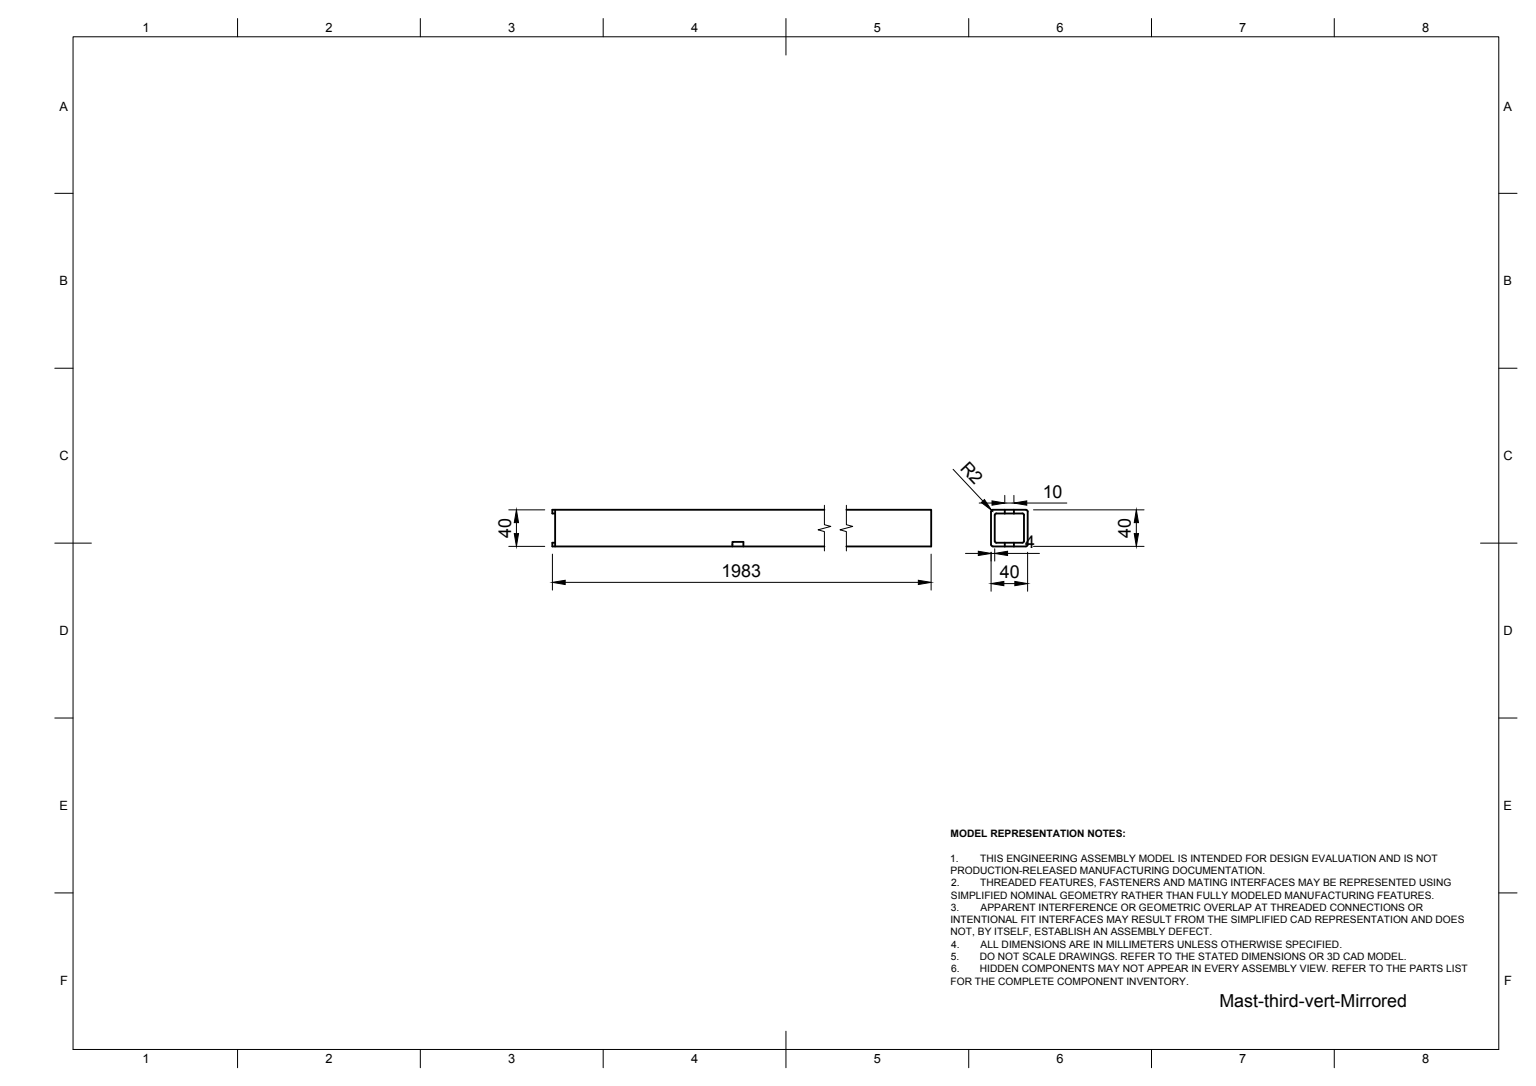
ISO-10303-21;
HEADER;
/* Generated by software containing ST-Developer
 * from STEP Tools, Inc. (www.steptools.com) 
 */

FILE_DESCRIPTION(
/* description */ (''),
/* implementation_level */ '2;1');

FILE_NAME(
/* name */ 'Mast-third-vert-Mirrored.step',
/* time_stamp */ '2026-10-07T11:02:43-07:00',
/* author */ (''),
/* organization */ (''),
/* preprocessor_version */ 'ST-DEVELOPER v20.2',
/* originating_system */ 'Autodesk Translation Framework v15.15.0.0',
/* authorisation */ '');

FILE_SCHEMA (('AUTOMOTIVE_DESIGN { 1 0 10303 214 3 1 1 }'));
ENDSEC;

DATA;
#10=MECHANICAL_DESIGN_GEOMETRIC_PRESENTATION_REPRESENTATION('',(#70),#5505);
#56=SHAPE_REPRESENTATION_RELATIONSHIP('SRR','None',#5541,#63);
#63=ADVANCED_BREP_SHAPE_REPRESENTATION('',(#77),#5502);
#70=STYLED_ITEM('',(#5585),#77);
#77=MANIFOLD_SOLID_BREP('Body1',#3297);
#102=FACE_BOUND('',#532,.T.);
#133=CYLINDRICAL_SURFACE('',#3531,2.);
#134=CYLINDRICAL_SURFACE('',#3535,2.);
#135=CYLINDRICAL_SURFACE('',#3538,1.8);
#136=CYLINDRICAL_SURFACE('',#3541,1.8);
#137=CYLINDRICAL_SURFACE('',#3544,1.8);
#138=CYLINDRICAL_SURFACE('',#3547,1.8);
#139=CYLINDRICAL_SURFACE('',#3553,2.);
#140=CYLINDRICAL_SURFACE('',#3556,2.);
#141=CYLINDRICAL_SURFACE('',#3558,2.);
#142=CYLINDRICAL_SURFACE('',#3559,2.);
#196=CIRCLE('',#3521,1.8);
#197=CIRCLE('',#3522,1.8);
#198=CIRCLE('',#3523,2.);
#199=CIRCLE('',#3524,2.);
#200=CIRCLE('',#3526,2.);
#201=CIRCLE('',#3527,2.);
#202=CIRCLE('',#3528,1.8);
#203=CIRCLE('',#3529,1.8);
#204=CIRCLE('',#3532,2.);
#205=CIRCLE('',#3533,2.);
#206=CIRCLE('',#3536,2.);
#207=CIRCLE('',#3539,1.8);
#208=CIRCLE('',#3542,1.8);
#209=CIRCLE('',#3545,1.8);
#210=CIRCLE('',#3548,1.8);
#211=CIRCLE('',#3550,2.);
#212=CIRCLE('',#3551,2.);
#213=CIRCLE('',#3552,2.);
#214=CIRCLE('',#3554,2.);
#215=CIRCLE('',#3560,2.);
#329=FACE_OUTER_BOUND('',#517,.T.);
#330=FACE_OUTER_BOUND('',#518,.T.);
#331=FACE_OUTER_BOUND('',#519,.T.);
#332=FACE_OUTER_BOUND('',#520,.T.);
#333=FACE_OUTER_BOUND('',#521,.T.);
#334=FACE_OUTER_BOUND('',#522,.T.);
#335=FACE_OUTER_BOUND('',#523,.T.);
#336=FACE_OUTER_BOUND('',#524,.T.);
#337=FACE_OUTER_BOUND('',#525,.T.);
#338=FACE_OUTER_BOUND('',#526,.T.);
#339=FACE_OUTER_BOUND('',#527,.T.);
#340=FACE_OUTER_BOUND('',#528,.T.);
#341=FACE_OUTER_BOUND('',#529,.T.);
#342=FACE_OUTER_BOUND('',#530,.T.);
#343=FACE_OUTER_BOUND('',#531,.T.);
#344=FACE_OUTER_BOUND('',#533,.T.);
#345=FACE_OUTER_BOUND('',#534,.T.);
#346=FACE_OUTER_BOUND('',#535,.T.);
#347=FACE_OUTER_BOUND('',#536,.T.);
#348=FACE_OUTER_BOUND('',#537,.T.);
#349=FACE_OUTER_BOUND('',#538,.T.);
#350=FACE_OUTER_BOUND('',#539,.T.);
#351=FACE_OUTER_BOUND('',#540,.T.);
#352=FACE_OUTER_BOUND('',#541,.T.);
#353=FACE_OUTER_BOUND('',#542,.T.);
#354=FACE_OUTER_BOUND('',#543,.T.);
#355=FACE_OUTER_BOUND('',#544,.T.);
#356=FACE_OUTER_BOUND('',#545,.T.);
#357=FACE_OUTER_BOUND('',#546,.T.);
#358=FACE_OUTER_BOUND('',#547,.T.);
#359=FACE_OUTER_BOUND('',#548,.T.);
#360=FACE_OUTER_BOUND('',#549,.T.);
#361=FACE_OUTER_BOUND('',#550,.T.);
#362=FACE_OUTER_BOUND('',#551,.T.);
#363=FACE_OUTER_BOUND('',#552,.T.);
#517=EDGE_LOOP('',(#2606,#2607,#2608,#2609,#2610,#2611,#2612,#2613,#2614,
#2615,#2616,#2617));
#518=EDGE_LOOP('',(#2618,#2619,#2620,#2621,#2622,#2623,#2624,#2625,#2626,
#2627,#2628,#2629));
#519=EDGE_LOOP('',(#2630,#2631,#2632,#2633,#2634,#2635,#2636,#2637));
#520=EDGE_LOOP('',(#2638,#2639,#2640,#2641));
#521=EDGE_LOOP('',(#2642,#2643,#2644,#2645,#2646,#2647,#2648,#2649,#2650,
#2651,#2652,#2653,#2654,#2655,#2656,#2657));
#522=EDGE_LOOP('',(#2658,#2659,#2660,#2661));
#523=EDGE_LOOP('',(#2662,#2663,#2664,#2665,#2666,#2667,#2668,#2669));
#524=EDGE_LOOP('',(#2670,#2671,#2672,#2673));
#525=EDGE_LOOP('',(#2674,#2675,#2676,#2677));
#526=EDGE_LOOP('',(#2678,#2679,#2680,#2681));
#527=EDGE_LOOP('',(#2682,#2683,#2684,#2685,#2686,#2687,#2688,#2689));
#528=EDGE_LOOP('',(#2690,#2691,#2692,#2693));
#529=EDGE_LOOP('',(#2694,#2695,#2696,#2697));
#530=EDGE_LOOP('',(#2698,#2699,#2700,#2701));
#531=EDGE_LOOP('',(#2702,#2703,#2704,#2705,#2706,#2707,#2708,#2709));
#532=EDGE_LOOP('',(#2710,#2711,#2712,#2713,#2714,#2715,#2716,#2717));
#533=EDGE_LOOP('',(#2718,#2719,#2720,#2721));
#534=EDGE_LOOP('',(#2722,#2723,#2724,#2725,#2726,#2727,#2728,#2729));
#535=EDGE_LOOP('',(#2730,#2731,#2732,#2733));
#536=EDGE_LOOP('',(#2734,#2735,#2736,#2737,#2738,#2739,#2740,#2741));
#537=EDGE_LOOP('',(#2742,#2743,#2744,#2745));
#538=EDGE_LOOP('',(#2746,#2747,#2748,#2749));
#539=EDGE_LOOP('',(#2750,#2751,#2752,#2753,#2754));
#540=EDGE_LOOP('',(#2755,#2756,#2757,#2758));
#541=EDGE_LOOP('',(#2759,#2760,#2761,#2762,#2763));
#542=EDGE_LOOP('',(#2764,#2765,#2766,#2767));
#543=EDGE_LOOP('',(#2768,#2769,#2770,#2771,#2772));
#544=EDGE_LOOP('',(#2773,#2774,#2775,#2776));
#545=EDGE_LOOP('',(#2777,#2778,#2779,#2780,#2781));
#546=EDGE_LOOP('',(#2782,#2783,#2784,#2785));
#547=EDGE_LOOP('',(#2786,#2787,#2788,#2789));
#548=EDGE_LOOP('',(#2790,#2791,#2792,#2793));
#549=EDGE_LOOP('',(#2794,#2795,#2796,#2797));
#550=EDGE_LOOP('',(#2798,#2799,#2800,#2801));
#551=EDGE_LOOP('',(#2802,#2803,#2804,#2805));
#552=EDGE_LOOP('',(#2806,#2807,#2808,#2809));
#813=LINE('',#5076,#1183);
#814=LINE('',#5078,#1184);
#815=LINE('',#5082,#1185);
#816=LINE('',#5086,#1186);
#817=LINE('',#5088,#1187);
#818=LINE('',#5090,#1188);
#819=LINE('',#5094,#1189);
#820=LINE('',#5097,#1190);
#821=LINE('',#5101,#1191);
#822=LINE('',#5105,#1192);
#823=LINE('',#5109,#1193);
#824=LINE('',#5111,#1194);
#825=LINE('',#5113,#1195);
#826=LINE('',#5117,#1196);
#827=LINE('',#5121,#1197);
#828=LINE('',#5122,#1198);
#829=LINE('',#5126,#1199);
#830=LINE('',#5128,#1200);
#831=LINE('',#5129,#1201);
#832=LINE('',#5131,#1202);
#833=LINE('',#5133,#1203);
#834=LINE('',#5135,#1204);
#835=LINE('',#5136,#1205);
#836=LINE('',#5141,#1206);
#837=LINE('',#5145,#1207);
#838=LINE('',#5147,#1208);
#839=LINE('',#5149,#1209);
#840=LINE('',#5151,#1210);
#841=LINE('',#5153,#1211);
#842=LINE('',#5154,#1212);
#843=LINE('',#5156,#1213);
#844=LINE('',#5158,#1214);
#845=LINE('',#5159,#1215);
#846=LINE('',#5161,#1216);
#847=LINE('',#5163,#1217);
#848=LINE('',#5165,#1218);
#849=LINE('',#5166,#1219);
#850=LINE('',#5169,#1220);
#851=LINE('',#5173,#1221);
#852=LINE('',#5175,#1222);
#853=LINE('',#5177,#1223);
#854=LINE('',#5178,#1224);
#855=LINE('',#5180,#1225);
#856=LINE('',#5181,#1226);
#857=LINE('',#5184,#1227);
#858=LINE('',#5188,#1228);
#859=LINE('',#5189,#1229);
#860=LINE('',#5192,#1230);
#861=LINE('',#5196,#1231);
#862=LINE('',#5198,#1232);
#863=LINE('',#5200,#1233);
#864=LINE('',#5201,#1234);
#865=LINE('',#5202,#1235);
#866=LINE('',#5205,#1236);
#867=LINE('',#5209,#1237);
#868=LINE('',#5210,#1238);
#869=LINE('',#5216,#1239);
#870=LINE('',#5221,#1240);
#871=LINE('',#5226,#1241);
#872=LINE('',#5229,#1242);
#873=LINE('',#5230,#1243);
#874=LINE('',#5232,#1244);
#875=LINE('',#5233,#1245);
#876=LINE('',#5235,#1246);
#877=LINE('',#5237,#1247);
#878=LINE('',#5239,#1248);
#879=LINE('',#5241,#1249);
#880=LINE('',#5242,#1250);
#881=LINE('',#5248,#1251);
#882=LINE('',#5249,#1252);
#883=LINE('',#5252,#1253);
#884=LINE('',#5253,#1254);
#885=LINE('',#5255,#1255);
#886=LINE('',#5259,#1256);
#887=LINE('',#5260,#1257);
#888=LINE('',#5263,#1258);
#889=LINE('',#5264,#1259);
#890=LINE('',#5266,#1260);
#891=LINE('',#5269,#1261);
#892=LINE('',#5271,#1262);
#893=LINE('',#5274,#1263);
#894=LINE('',#5276,#1264);
#1183=VECTOR('',#4143,1000.);
#1184=VECTOR('',#4144,1000.);
#1185=VECTOR('',#4147,1000.);
#1186=VECTOR('',#4150,1000.);
#1187=VECTOR('',#4151,1000.);
#1188=VECTOR('',#4152,1000.);
#1189=VECTOR('',#4155,1000.);
#1190=VECTOR('',#4158,1000.);
#1191=VECTOR('',#4161,1000.);
#1192=VECTOR('',#4164,1000.);
#1193=VECTOR('',#4167,1000.);
#1194=VECTOR('',#4168,1000.);
#1195=VECTOR('',#4169,1000.);
#1196=VECTOR('',#4172,1000.);
#1197=VECTOR('',#4175,1000.);
#1198=VECTOR('',#4176,1000.);
#1199=VECTOR('',#4179,1000.);
#1200=VECTOR('',#4180,1000.);
#1201=VECTOR('',#4181,1000.);
#1202=VECTOR('',#4182,1000.);
#1203=VECTOR('',#4183,1000.);
#1204=VECTOR('',#4184,1000.);
#1205=VECTOR('',#4185,1000.);
#1206=VECTOR('',#4190,1000.);
#1207=VECTOR('',#4195,1000.);
#1208=VECTOR('',#4196,1000.);
#1209=VECTOR('',#4197,1000.);
#1210=VECTOR('',#4198,1000.);
#1211=VECTOR('',#4199,1000.);
#1212=VECTOR('',#4200,1000.);
#1213=VECTOR('',#4201,1000.);
#1214=VECTOR('',#4202,1000.);
#1215=VECTOR('',#4203,1000.);
#1216=VECTOR('',#4204,1000.);
#1217=VECTOR('',#4205,1000.);
#1218=VECTOR('',#4206,1000.);
#1219=VECTOR('',#4207,1000.);
#1220=VECTOR('',#4210,1000.);
#1221=VECTOR('',#4215,1000.);
#1222=VECTOR('',#4216,1000.);
#1223=VECTOR('',#4217,1000.);
#1224=VECTOR('',#4218,1000.);
#1225=VECTOR('',#4219,1000.);
#1226=VECTOR('',#4220,1000.);
#1227=VECTOR('',#4223,1000.);
#1228=VECTOR('',#4228,1000.);
#1229=VECTOR('',#4229,1000.);
#1230=VECTOR('',#4232,1000.);
#1231=VECTOR('',#4237,1000.);
#1232=VECTOR('',#4238,1000.);
#1233=VECTOR('',#4239,1000.);
#1234=VECTOR('',#4240,1000.);
#1235=VECTOR('',#4241,1000.);
#1236=VECTOR('',#4244,1000.);
#1237=VECTOR('',#4249,1000.);
#1238=VECTOR('',#4250,1000.);
#1239=VECTOR('',#4257,1000.);
#1240=VECTOR('',#4262,1000.);
#1241=VECTOR('',#4269,1000.);
#1242=VECTOR('',#4272,1000.);
#1243=VECTOR('',#4273,1000.);
#1244=VECTOR('',#4274,1000.);
#1245=VECTOR('',#4275,1000.);
#1246=VECTOR('',#4278,1000.);
#1247=VECTOR('',#4281,1000.);
#1248=VECTOR('',#4282,1000.);
#1249=VECTOR('',#4283,1000.);
#1250=VECTOR('',#4284,1000.);
#1251=VECTOR('',#4293,1000.);
#1252=VECTOR('',#4294,1000.);
#1253=VECTOR('',#4297,1000.);
#1254=VECTOR('',#4298,1000.);
#1255=VECTOR('',#4301,1000.);
#1256=VECTOR('',#4306,1000.);
#1257=VECTOR('',#4307,1000.);
#1258=VECTOR('',#4310,1000.);
#1259=VECTOR('',#4311,1000.);
#1260=VECTOR('',#4314,1000.);
#1261=VECTOR('',#4319,1000.);
#1262=VECTOR('',#4322,1000.);
#1263=VECTOR('',#4327,1000.);
#1264=VECTOR('',#4330,1000.);
#1511=VERTEX_POINT('',#5074);
#1512=VERTEX_POINT('',#5075);
#1513=VERTEX_POINT('',#5077);
#1514=VERTEX_POINT('',#5079);
#1515=VERTEX_POINT('',#5081);
#1516=VERTEX_POINT('',#5083);
#1517=VERTEX_POINT('',#5085);
#1518=VERTEX_POINT('',#5087);
#1519=VERTEX_POINT('',#5089);
#1520=VERTEX_POINT('',#5091);
#1521=VERTEX_POINT('',#5093);
#1522=VERTEX_POINT('',#5095);
#1523=VERTEX_POINT('',#5099);
#1524=VERTEX_POINT('',#5100);
#1525=VERTEX_POINT('',#5102);
#1526=VERTEX_POINT('',#5104);
#1527=VERTEX_POINT('',#5106);
#1528=VERTEX_POINT('',#5108);
#1529=VERTEX_POINT('',#5110);
#1530=VERTEX_POINT('',#5112);
#1531=VERTEX_POINT('',#5114);
#1532=VERTEX_POINT('',#5116);
#1533=VERTEX_POINT('',#5118);
#1534=VERTEX_POINT('',#5120);
#1535=VERTEX_POINT('',#5124);
#1536=VERTEX_POINT('',#5125);
#1537=VERTEX_POINT('',#5127);
#1538=VERTEX_POINT('',#5130);
#1539=VERTEX_POINT('',#5132);
#1540=VERTEX_POINT('',#5134);
#1541=VERTEX_POINT('',#5138);
#1542=VERTEX_POINT('',#5140);
#1543=VERTEX_POINT('',#5144);
#1544=VERTEX_POINT('',#5146);
#1545=VERTEX_POINT('',#5148);
#1546=VERTEX_POINT('',#5150);
#1547=VERTEX_POINT('',#5152);
#1548=VERTEX_POINT('',#5155);
#1549=VERTEX_POINT('',#5157);
#1550=VERTEX_POINT('',#5160);
#1551=VERTEX_POINT('',#5162);
#1552=VERTEX_POINT('',#5164);
#1553=VERTEX_POINT('',#5168);
#1554=VERTEX_POINT('',#5172);
#1555=VERTEX_POINT('',#5174);
#1556=VERTEX_POINT('',#5176);
#1557=VERTEX_POINT('',#5179);
#1558=VERTEX_POINT('',#5183);
#1559=VERTEX_POINT('',#5187);
#1560=VERTEX_POINT('',#5191);
#1561=VERTEX_POINT('',#5195);
#1562=VERTEX_POINT('',#5197);
#1563=VERTEX_POINT('',#5199);
#1564=VERTEX_POINT('',#5204);
#1565=VERTEX_POINT('',#5208);
#1566=VERTEX_POINT('',#5214);
#1567=VERTEX_POINT('',#5215);
#1568=VERTEX_POINT('',#5218);
#1569=VERTEX_POINT('',#5220);
#1570=VERTEX_POINT('',#5224);
#1571=VERTEX_POINT('',#5228);
#1572=VERTEX_POINT('',#5231);
#1573=VERTEX_POINT('',#5238);
#1574=VERTEX_POINT('',#5240);
#1575=VERTEX_POINT('',#5247);
#1576=VERTEX_POINT('',#5251);
#1577=VERTEX_POINT('',#5258);
#1578=VERTEX_POINT('',#5262);
#1898=EDGE_CURVE('',#1511,#1512,#813,.T.);
#1899=EDGE_CURVE('',#1512,#1513,#814,.T.);
#1900=EDGE_CURVE('',#1514,#1513,#196,.T.);
#1901=EDGE_CURVE('',#1515,#1514,#815,.T.);
#1902=EDGE_CURVE('',#1516,#1515,#197,.T.);
#1903=EDGE_CURVE('',#1517,#1516,#816,.T.);
#1904=EDGE_CURVE('',#1517,#1518,#817,.T.);
#1905=EDGE_CURVE('',#1518,#1519,#818,.T.);
#1906=EDGE_CURVE('',#1519,#1520,#198,.T.);
#1907=EDGE_CURVE('',#1520,#1521,#819,.T.);
#1908=EDGE_CURVE('',#1521,#1522,#199,.T.);
#1909=EDGE_CURVE('',#1522,#1511,#820,.F.);
#1910=EDGE_CURVE('',#1523,#1524,#821,.F.);
#1911=EDGE_CURVE('',#1524,#1525,#200,.T.);
#1912=EDGE_CURVE('',#1525,#1526,#822,.F.);
#1913=EDGE_CURVE('',#1526,#1527,#201,.T.);
#1914=EDGE_CURVE('',#1527,#1528,#823,.T.);
#1915=EDGE_CURVE('',#1529,#1528,#824,.T.);
#1916=EDGE_CURVE('',#1530,#1529,#825,.T.);
#1917=EDGE_CURVE('',#1531,#1530,#202,.T.);
#1918=EDGE_CURVE('',#1531,#1532,#826,.T.);
#1919=EDGE_CURVE('',#1533,#1532,#203,.T.);
#1920=EDGE_CURVE('',#1533,#1534,#827,.T.);
#1921=EDGE_CURVE('',#1523,#1534,#828,.T.);
#1922=EDGE_CURVE('',#1535,#1536,#829,.T.);
#1923=EDGE_CURVE('',#1535,#1537,#830,.T.);
#1924=EDGE_CURVE('',#1526,#1537,#831,.T.);
#1925=EDGE_CURVE('',#1525,#1538,#832,.T.);
#1926=EDGE_CURVE('',#1538,#1539,#833,.T.);
#1927=EDGE_CURVE('',#1540,#1539,#834,.T.);
#1928=EDGE_CURVE('',#1536,#1540,#835,.T.);
#1929=EDGE_CURVE('',#1539,#1541,#204,.T.);
#1930=EDGE_CURVE('',#1542,#1541,#836,.T.);
#1931=EDGE_CURVE('',#1540,#1542,#205,.F.);
#1932=EDGE_CURVE('',#1541,#1543,#837,.T.);
#1933=EDGE_CURVE('',#1544,#1543,#838,.T.);
#1934=EDGE_CURVE('',#1544,#1545,#839,.T.);
#1935=EDGE_CURVE('',#1545,#1546,#840,.T.);
#1936=EDGE_CURVE('',#1547,#1546,#841,.T.);
#1937=EDGE_CURVE('',#1519,#1547,#842,.T.);
#1938=EDGE_CURVE('',#1548,#1518,#843,.T.);
#1939=EDGE_CURVE('',#1548,#1549,#844,.T.);
#1940=EDGE_CURVE('',#1549,#1528,#845,.T.);
#1941=EDGE_CURVE('',#1527,#1550,#846,.T.);
#1942=EDGE_CURVE('',#1550,#1551,#847,.T.);
#1943=EDGE_CURVE('',#1552,#1551,#848,.T.);
#1944=EDGE_CURVE('',#1542,#1552,#849,.T.);
#1945=EDGE_CURVE('',#1520,#1553,#850,.T.);
#1946=EDGE_CURVE('',#1553,#1547,#206,.F.);
#1947=EDGE_CURVE('',#1513,#1554,#851,.T.);
#1948=EDGE_CURVE('',#1555,#1512,#852,.T.);
#1949=EDGE_CURVE('',#1555,#1556,#853,.T.);
#1950=EDGE_CURVE('',#1556,#1534,#854,.T.);
#1951=EDGE_CURVE('',#1533,#1557,#855,.T.);
#1952=EDGE_CURVE('',#1557,#1554,#856,.T.);
#1953=EDGE_CURVE('',#1514,#1558,#857,.T.);
#1954=EDGE_CURVE('',#1558,#1554,#207,.T.);
#1955=EDGE_CURVE('',#1515,#1559,#858,.T.);
#1956=EDGE_CURVE('',#1559,#1558,#859,.T.);
#1957=EDGE_CURVE('',#1516,#1560,#860,.T.);
#1958=EDGE_CURVE('',#1560,#1559,#208,.T.);
#1959=EDGE_CURVE('',#1530,#1561,#861,.T.);
#1960=EDGE_CURVE('',#1562,#1529,#862,.T.);
#1961=EDGE_CURVE('',#1563,#1562,#863,.T.);
#1962=EDGE_CURVE('',#1563,#1517,#864,.T.);
#1963=EDGE_CURVE('',#1561,#1560,#865,.T.);
#1964=EDGE_CURVE('',#1531,#1564,#866,.T.);
#1965=EDGE_CURVE('',#1564,#1561,#209,.T.);
#1966=EDGE_CURVE('',#1532,#1565,#867,.T.);
#1967=EDGE_CURVE('',#1564,#1565,#868,.T.);
#1968=EDGE_CURVE('',#1557,#1565,#210,.T.);
#1969=EDGE_CURVE('',#1566,#1567,#869,.T.);
#1970=EDGE_CURVE('',#1543,#1566,#211,.T.);
#1971=EDGE_CURVE('',#1568,#1538,#212,.T.);
#1972=EDGE_CURVE('',#1569,#1568,#870,.T.);
#1973=EDGE_CURVE('',#1567,#1569,#213,.T.);
#1974=EDGE_CURVE('',#1570,#1544,#214,.F.);
#1975=EDGE_CURVE('',#1570,#1566,#871,.T.);
#1976=EDGE_CURVE('',#1571,#1570,#872,.T.);
#1977=EDGE_CURVE('',#1521,#1567,#873,.T.);
#1978=EDGE_CURVE('',#1572,#1553,#874,.T.);
#1979=EDGE_CURVE('',#1572,#1571,#875,.T.);
#1980=EDGE_CURVE('',#1522,#1569,#876,.T.);
#1981=EDGE_CURVE('',#1524,#1568,#877,.T.);
#1982=EDGE_CURVE('',#1573,#1523,#878,.T.);
#1983=EDGE_CURVE('',#1574,#1573,#879,.T.);
#1984=EDGE_CURVE('',#1574,#1511,#880,.T.);
#1985=EDGE_CURVE('',#1537,#1550,#215,.F.);
#1986=EDGE_CURVE('',#1575,#1571,#881,.T.);
#1987=EDGE_CURVE('',#1575,#1545,#882,.T.);
#1988=EDGE_CURVE('',#1576,#1572,#883,.T.);
#1989=EDGE_CURVE('',#1576,#1575,#884,.T.);
#1990=EDGE_CURVE('',#1576,#1546,#885,.T.);
#1991=EDGE_CURVE('',#1577,#1552,#886,.T.);
#1992=EDGE_CURVE('',#1577,#1536,#887,.T.);
#1993=EDGE_CURVE('',#1578,#1577,#888,.T.);
#1994=EDGE_CURVE('',#1578,#1535,#889,.T.);
#1995=EDGE_CURVE('',#1578,#1551,#890,.T.);
#1996=EDGE_CURVE('',#1563,#1548,#891,.T.);
#1997=EDGE_CURVE('',#1562,#1549,#892,.T.);
#1998=EDGE_CURVE('',#1574,#1555,#893,.T.);
#1999=EDGE_CURVE('',#1573,#1556,#894,.T.);
#2606=ORIENTED_EDGE('',*,*,#1898,.T.);
#2607=ORIENTED_EDGE('',*,*,#1899,.T.);
#2608=ORIENTED_EDGE('',*,*,#1900,.F.);
#2609=ORIENTED_EDGE('',*,*,#1901,.F.);
#2610=ORIENTED_EDGE('',*,*,#1902,.F.);
#2611=ORIENTED_EDGE('',*,*,#1903,.F.);
#2612=ORIENTED_EDGE('',*,*,#1904,.T.);
#2613=ORIENTED_EDGE('',*,*,#1905,.T.);
#2614=ORIENTED_EDGE('',*,*,#1906,.T.);
#2615=ORIENTED_EDGE('',*,*,#1907,.T.);
#2616=ORIENTED_EDGE('',*,*,#1908,.T.);
#2617=ORIENTED_EDGE('',*,*,#1909,.T.);
#2618=ORIENTED_EDGE('',*,*,#1910,.T.);
#2619=ORIENTED_EDGE('',*,*,#1911,.T.);
#2620=ORIENTED_EDGE('',*,*,#1912,.T.);
#2621=ORIENTED_EDGE('',*,*,#1913,.T.);
#2622=ORIENTED_EDGE('',*,*,#1914,.T.);
#2623=ORIENTED_EDGE('',*,*,#1915,.F.);
#2624=ORIENTED_EDGE('',*,*,#1916,.F.);
#2625=ORIENTED_EDGE('',*,*,#1917,.F.);
#2626=ORIENTED_EDGE('',*,*,#1918,.T.);
#2627=ORIENTED_EDGE('',*,*,#1919,.F.);
#2628=ORIENTED_EDGE('',*,*,#1920,.T.);
#2629=ORIENTED_EDGE('',*,*,#1921,.F.);
#2630=ORIENTED_EDGE('',*,*,#1922,.F.);
#2631=ORIENTED_EDGE('',*,*,#1923,.T.);
#2632=ORIENTED_EDGE('',*,*,#1924,.F.);
#2633=ORIENTED_EDGE('',*,*,#1912,.F.);
#2634=ORIENTED_EDGE('',*,*,#1925,.T.);
#2635=ORIENTED_EDGE('',*,*,#1926,.T.);
#2636=ORIENTED_EDGE('',*,*,#1927,.F.);
#2637=ORIENTED_EDGE('',*,*,#1928,.F.);
#2638=ORIENTED_EDGE('',*,*,#1927,.T.);
#2639=ORIENTED_EDGE('',*,*,#1929,.T.);
#2640=ORIENTED_EDGE('',*,*,#1930,.F.);
#2641=ORIENTED_EDGE('',*,*,#1931,.F.);
#2642=ORIENTED_EDGE('',*,*,#1930,.T.);
#2643=ORIENTED_EDGE('',*,*,#1932,.T.);
#2644=ORIENTED_EDGE('',*,*,#1933,.F.);
#2645=ORIENTED_EDGE('',*,*,#1934,.T.);
#2646=ORIENTED_EDGE('',*,*,#1935,.T.);
#2647=ORIENTED_EDGE('',*,*,#1936,.F.);
#2648=ORIENTED_EDGE('',*,*,#1937,.F.);
#2649=ORIENTED_EDGE('',*,*,#1905,.F.);
#2650=ORIENTED_EDGE('',*,*,#1938,.F.);
#2651=ORIENTED_EDGE('',*,*,#1939,.T.);
#2652=ORIENTED_EDGE('',*,*,#1940,.T.);
#2653=ORIENTED_EDGE('',*,*,#1914,.F.);
#2654=ORIENTED_EDGE('',*,*,#1941,.T.);
#2655=ORIENTED_EDGE('',*,*,#1942,.T.);
#2656=ORIENTED_EDGE('',*,*,#1943,.F.);
#2657=ORIENTED_EDGE('',*,*,#1944,.F.);
#2658=ORIENTED_EDGE('',*,*,#1945,.F.);
#2659=ORIENTED_EDGE('',*,*,#1906,.F.);
#2660=ORIENTED_EDGE('',*,*,#1937,.T.);
#2661=ORIENTED_EDGE('',*,*,#1946,.F.);
#2662=ORIENTED_EDGE('',*,*,#1947,.F.);
#2663=ORIENTED_EDGE('',*,*,#1899,.F.);
#2664=ORIENTED_EDGE('',*,*,#1948,.F.);
#2665=ORIENTED_EDGE('',*,*,#1949,.T.);
#2666=ORIENTED_EDGE('',*,*,#1950,.T.);
#2667=ORIENTED_EDGE('',*,*,#1920,.F.);
#2668=ORIENTED_EDGE('',*,*,#1951,.T.);
#2669=ORIENTED_EDGE('',*,*,#1952,.T.);
#2670=ORIENTED_EDGE('',*,*,#1953,.F.);
#2671=ORIENTED_EDGE('',*,*,#1900,.T.);
#2672=ORIENTED_EDGE('',*,*,#1947,.T.);
#2673=ORIENTED_EDGE('',*,*,#1954,.F.);
#2674=ORIENTED_EDGE('',*,*,#1955,.F.);
#2675=ORIENTED_EDGE('',*,*,#1901,.T.);
#2676=ORIENTED_EDGE('',*,*,#1953,.T.);
#2677=ORIENTED_EDGE('',*,*,#1956,.F.);
#2678=ORIENTED_EDGE('',*,*,#1957,.F.);
#2679=ORIENTED_EDGE('',*,*,#1902,.T.);
#2680=ORIENTED_EDGE('',*,*,#1955,.T.);
#2681=ORIENTED_EDGE('',*,*,#1958,.F.);
#2682=ORIENTED_EDGE('',*,*,#1959,.F.);
#2683=ORIENTED_EDGE('',*,*,#1916,.T.);
#2684=ORIENTED_EDGE('',*,*,#1960,.F.);
#2685=ORIENTED_EDGE('',*,*,#1961,.F.);
#2686=ORIENTED_EDGE('',*,*,#1962,.T.);
#2687=ORIENTED_EDGE('',*,*,#1903,.T.);
#2688=ORIENTED_EDGE('',*,*,#1957,.T.);
#2689=ORIENTED_EDGE('',*,*,#1963,.F.);
#2690=ORIENTED_EDGE('',*,*,#1964,.F.);
#2691=ORIENTED_EDGE('',*,*,#1917,.T.);
#2692=ORIENTED_EDGE('',*,*,#1959,.T.);
#2693=ORIENTED_EDGE('',*,*,#1965,.F.);
#2694=ORIENTED_EDGE('',*,*,#1966,.F.);
#2695=ORIENTED_EDGE('',*,*,#1918,.F.);
#2696=ORIENTED_EDGE('',*,*,#1964,.T.);
#2697=ORIENTED_EDGE('',*,*,#1967,.T.);
#2698=ORIENTED_EDGE('',*,*,#1968,.F.);
#2699=ORIENTED_EDGE('',*,*,#1951,.F.);
#2700=ORIENTED_EDGE('',*,*,#1919,.T.);
#2701=ORIENTED_EDGE('',*,*,#1966,.T.);
#2702=ORIENTED_EDGE('',*,*,#1969,.F.);
#2703=ORIENTED_EDGE('',*,*,#1970,.F.);
#2704=ORIENTED_EDGE('',*,*,#1932,.F.);
#2705=ORIENTED_EDGE('',*,*,#1929,.F.);
#2706=ORIENTED_EDGE('',*,*,#1926,.F.);
#2707=ORIENTED_EDGE('',*,*,#1971,.F.);
#2708=ORIENTED_EDGE('',*,*,#1972,.F.);
#2709=ORIENTED_EDGE('',*,*,#1973,.F.);
#2710=ORIENTED_EDGE('',*,*,#1954,.T.);
#2711=ORIENTED_EDGE('',*,*,#1952,.F.);
#2712=ORIENTED_EDGE('',*,*,#1968,.T.);
#2713=ORIENTED_EDGE('',*,*,#1967,.F.);
#2714=ORIENTED_EDGE('',*,*,#1965,.T.);
#2715=ORIENTED_EDGE('',*,*,#1963,.T.);
#2716=ORIENTED_EDGE('',*,*,#1958,.T.);
#2717=ORIENTED_EDGE('',*,*,#1956,.T.);
#2718=ORIENTED_EDGE('',*,*,#1974,.T.);
#2719=ORIENTED_EDGE('',*,*,#1933,.T.);
#2720=ORIENTED_EDGE('',*,*,#1970,.T.);
#2721=ORIENTED_EDGE('',*,*,#1975,.F.);
#2722=ORIENTED_EDGE('',*,*,#1976,.T.);
#2723=ORIENTED_EDGE('',*,*,#1975,.T.);
#2724=ORIENTED_EDGE('',*,*,#1969,.T.);
#2725=ORIENTED_EDGE('',*,*,#1977,.F.);
#2726=ORIENTED_EDGE('',*,*,#1907,.F.);
#2727=ORIENTED_EDGE('',*,*,#1945,.T.);
#2728=ORIENTED_EDGE('',*,*,#1978,.F.);
#2729=ORIENTED_EDGE('',*,*,#1979,.T.);
#2730=ORIENTED_EDGE('',*,*,#1980,.F.);
#2731=ORIENTED_EDGE('',*,*,#1908,.F.);
#2732=ORIENTED_EDGE('',*,*,#1977,.T.);
#2733=ORIENTED_EDGE('',*,*,#1973,.T.);
#2734=ORIENTED_EDGE('',*,*,#1981,.F.);
#2735=ORIENTED_EDGE('',*,*,#1910,.F.);
#2736=ORIENTED_EDGE('',*,*,#1982,.F.);
#2737=ORIENTED_EDGE('',*,*,#1983,.F.);
#2738=ORIENTED_EDGE('',*,*,#1984,.T.);
#2739=ORIENTED_EDGE('',*,*,#1909,.F.);
#2740=ORIENTED_EDGE('',*,*,#1980,.T.);
#2741=ORIENTED_EDGE('',*,*,#1972,.T.);
#2742=ORIENTED_EDGE('',*,*,#1925,.F.);
#2743=ORIENTED_EDGE('',*,*,#1911,.F.);
#2744=ORIENTED_EDGE('',*,*,#1981,.T.);
#2745=ORIENTED_EDGE('',*,*,#1971,.T.);
#2746=ORIENTED_EDGE('',*,*,#1985,.T.);
#2747=ORIENTED_EDGE('',*,*,#1941,.F.);
#2748=ORIENTED_EDGE('',*,*,#1913,.F.);
#2749=ORIENTED_EDGE('',*,*,#1924,.T.);
#2750=ORIENTED_EDGE('',*,*,#1974,.F.);
#2751=ORIENTED_EDGE('',*,*,#1976,.F.);
#2752=ORIENTED_EDGE('',*,*,#1986,.F.);
#2753=ORIENTED_EDGE('',*,*,#1987,.T.);
#2754=ORIENTED_EDGE('',*,*,#1934,.F.);
#2755=ORIENTED_EDGE('',*,*,#1979,.F.);
#2756=ORIENTED_EDGE('',*,*,#1988,.F.);
#2757=ORIENTED_EDGE('',*,*,#1989,.T.);
#2758=ORIENTED_EDGE('',*,*,#1986,.T.);
#2759=ORIENTED_EDGE('',*,*,#1978,.T.);
#2760=ORIENTED_EDGE('',*,*,#1946,.T.);
#2761=ORIENTED_EDGE('',*,*,#1936,.T.);
#2762=ORIENTED_EDGE('',*,*,#1990,.F.);
#2763=ORIENTED_EDGE('',*,*,#1988,.T.);
#2764=ORIENTED_EDGE('',*,*,#1935,.F.);
#2765=ORIENTED_EDGE('',*,*,#1987,.F.);
#2766=ORIENTED_EDGE('',*,*,#1989,.F.);
#2767=ORIENTED_EDGE('',*,*,#1990,.T.);
#2768=ORIENTED_EDGE('',*,*,#1928,.T.);
#2769=ORIENTED_EDGE('',*,*,#1931,.T.);
#2770=ORIENTED_EDGE('',*,*,#1944,.T.);
#2771=ORIENTED_EDGE('',*,*,#1991,.F.);
#2772=ORIENTED_EDGE('',*,*,#1992,.T.);
#2773=ORIENTED_EDGE('',*,*,#1922,.T.);
#2774=ORIENTED_EDGE('',*,*,#1992,.F.);
#2775=ORIENTED_EDGE('',*,*,#1993,.F.);
#2776=ORIENTED_EDGE('',*,*,#1994,.T.);
#2777=ORIENTED_EDGE('',*,*,#1985,.F.);
#2778=ORIENTED_EDGE('',*,*,#1923,.F.);
#2779=ORIENTED_EDGE('',*,*,#1994,.F.);
#2780=ORIENTED_EDGE('',*,*,#1995,.T.);
#2781=ORIENTED_EDGE('',*,*,#1942,.F.);
#2782=ORIENTED_EDGE('',*,*,#1991,.T.);
#2783=ORIENTED_EDGE('',*,*,#1943,.T.);
#2784=ORIENTED_EDGE('',*,*,#1995,.F.);
#2785=ORIENTED_EDGE('',*,*,#1993,.T.);
#2786=ORIENTED_EDGE('',*,*,#1904,.F.);
#2787=ORIENTED_EDGE('',*,*,#1962,.F.);
#2788=ORIENTED_EDGE('',*,*,#1996,.T.);
#2789=ORIENTED_EDGE('',*,*,#1938,.T.);
#2790=ORIENTED_EDGE('',*,*,#1915,.T.);
#2791=ORIENTED_EDGE('',*,*,#1940,.F.);
#2792=ORIENTED_EDGE('',*,*,#1997,.F.);
#2793=ORIENTED_EDGE('',*,*,#1960,.T.);
#2794=ORIENTED_EDGE('',*,*,#1996,.F.);
#2795=ORIENTED_EDGE('',*,*,#1961,.T.);
#2796=ORIENTED_EDGE('',*,*,#1997,.T.);
#2797=ORIENTED_EDGE('',*,*,#1939,.F.);
#2798=ORIENTED_EDGE('',*,*,#1898,.F.);
#2799=ORIENTED_EDGE('',*,*,#1984,.F.);
#2800=ORIENTED_EDGE('',*,*,#1998,.T.);
#2801=ORIENTED_EDGE('',*,*,#1948,.T.);
#2802=ORIENTED_EDGE('',*,*,#1921,.T.);
#2803=ORIENTED_EDGE('',*,*,#1950,.F.);
#2804=ORIENTED_EDGE('',*,*,#1999,.F.);
#2805=ORIENTED_EDGE('',*,*,#1982,.T.);
#2806=ORIENTED_EDGE('',*,*,#1998,.F.);
#2807=ORIENTED_EDGE('',*,*,#1983,.T.);
#2808=ORIENTED_EDGE('',*,*,#1999,.T.);
#2809=ORIENTED_EDGE('',*,*,#1949,.F.);
#3074=PLANE('',#3520);
#3075=PLANE('',#3525);
#3076=PLANE('',#3530);
#3077=PLANE('',#3534);
#3078=PLANE('',#3537);
#3079=PLANE('',#3540);
#3080=PLANE('',#3543);
#3081=PLANE('',#3546);
#3082=PLANE('',#3549);
#3083=PLANE('',#3555);
#3084=PLANE('',#3557);
#3085=PLANE('',#3561);
#3086=PLANE('',#3562);
#3087=PLANE('',#3563);
#3088=PLANE('',#3564);
#3089=PLANE('',#3565);
#3090=PLANE('',#3566);
#3091=PLANE('',#3567);
#3092=PLANE('',#3568);
#3093=PLANE('',#3569);
#3094=PLANE('',#3570);
#3095=PLANE('',#3571);
#3096=PLANE('',#3572);
#3097=PLANE('',#3573);
#3098=PLANE('',#3574);
#3220=ADVANCED_FACE('',(#329),#3074,.F.);
#3221=ADVANCED_FACE('',(#330),#3075,.F.);
#3222=ADVANCED_FACE('',(#331),#3076,.T.);
#3223=ADVANCED_FACE('',(#332),#133,.T.);
#3224=ADVANCED_FACE('',(#333),#3077,.T.);
#3225=ADVANCED_FACE('',(#334),#134,.T.);
#3226=ADVANCED_FACE('',(#335),#3078,.T.);
#3227=ADVANCED_FACE('',(#336),#135,.F.);
#3228=ADVANCED_FACE('',(#337),#3079,.T.);
#3229=ADVANCED_FACE('',(#338),#136,.F.);
#3230=ADVANCED_FACE('',(#339),#3080,.T.);
#3231=ADVANCED_FACE('',(#340),#137,.F.);
#3232=ADVANCED_FACE('',(#341),#3081,.T.);
#3233=ADVANCED_FACE('',(#342),#138,.F.);
#3234=ADVANCED_FACE('',(#343,#102),#3082,.T.);
#3235=ADVANCED_FACE('',(#344),#139,.T.);
#3236=ADVANCED_FACE('',(#345),#3083,.T.);
#3237=ADVANCED_FACE('',(#346),#140,.T.);
#3238=ADVANCED_FACE('',(#347),#3084,.T.);
#3239=ADVANCED_FACE('',(#348),#141,.T.);
#3240=ADVANCED_FACE('',(#349),#142,.T.);
#3241=ADVANCED_FACE('',(#350),#3085,.F.);
#3242=ADVANCED_FACE('',(#351),#3086,.F.);
#3243=ADVANCED_FACE('',(#352),#3087,.T.);
#3244=ADVANCED_FACE('',(#353),#3088,.F.);
#3245=ADVANCED_FACE('',(#354),#3089,.T.);
#3246=ADVANCED_FACE('',(#355),#3090,.T.);
#3247=ADVANCED_FACE('',(#356),#3091,.F.);
#3248=ADVANCED_FACE('',(#357),#3092,.T.);
#3249=ADVANCED_FACE('',(#358),#3093,.F.);
#3250=ADVANCED_FACE('',(#359),#3094,.T.);
#3251=ADVANCED_FACE('',(#360),#3095,.F.);
#3252=ADVANCED_FACE('',(#361),#3096,.F.);
#3253=ADVANCED_FACE('',(#362),#3097,.T.);
#3254=ADVANCED_FACE('',(#363),#3098,.F.);
#3297=CLOSED_SHELL('',(#3220,#3221,#3222,#3223,#3224,#3225,#3226,#3227,
#3228,#3229,#3230,#3231,#3232,#3233,#3234,#3235,#3236,#3237,#3238,#3239,
#3240,#3241,#3242,#3243,#3244,#3245,#3246,#3247,#3248,#3249,#3250,#3251,
#3252,#3253,#3254));
#3519=AXIS2_PLACEMENT_3D('',#5072,#4139,#4140);
#3520=AXIS2_PLACEMENT_3D('',#5073,#4141,#4142);
#3521=AXIS2_PLACEMENT_3D('',#5080,#4145,#4146);
#3522=AXIS2_PLACEMENT_3D('',#5084,#4148,#4149);
#3523=AXIS2_PLACEMENT_3D('',#5092,#4153,#4154);
#3524=AXIS2_PLACEMENT_3D('',#5096,#4156,#4157);
#3525=AXIS2_PLACEMENT_3D('',#5098,#4159,#4160);
#3526=AXIS2_PLACEMENT_3D('',#5103,#4162,#4163);
#3527=AXIS2_PLACEMENT_3D('',#5107,#4165,#4166);
#3528=AXIS2_PLACEMENT_3D('',#5115,#4170,#4171);
#3529=AXIS2_PLACEMENT_3D('',#5119,#4173,#4174);
#3530=AXIS2_PLACEMENT_3D('',#5123,#4177,#4178);
#3531=AXIS2_PLACEMENT_3D('',#5137,#4186,#4187);
#3532=AXIS2_PLACEMENT_3D('',#5139,#4188,#4189);
#3533=AXIS2_PLACEMENT_3D('',#5142,#4191,#4192);
#3534=AXIS2_PLACEMENT_3D('',#5143,#4193,#4194);
#3535=AXIS2_PLACEMENT_3D('',#5167,#4208,#4209);
#3536=AXIS2_PLACEMENT_3D('',#5170,#4211,#4212);
#3537=AXIS2_PLACEMENT_3D('',#5171,#4213,#4214);
#3538=AXIS2_PLACEMENT_3D('',#5182,#4221,#4222);
#3539=AXIS2_PLACEMENT_3D('',#5185,#4224,#4225);
#3540=AXIS2_PLACEMENT_3D('',#5186,#4226,#4227);
#3541=AXIS2_PLACEMENT_3D('',#5190,#4230,#4231);
#3542=AXIS2_PLACEMENT_3D('',#5193,#4233,#4234);
#3543=AXIS2_PLACEMENT_3D('',#5194,#4235,#4236);
#3544=AXIS2_PLACEMENT_3D('',#5203,#4242,#4243);
#3545=AXIS2_PLACEMENT_3D('',#5206,#4245,#4246);
#3546=AXIS2_PLACEMENT_3D('',#5207,#4247,#4248);
#3547=AXIS2_PLACEMENT_3D('',#5211,#4251,#4252);
#3548=AXIS2_PLACEMENT_3D('',#5212,#4253,#4254);
#3549=AXIS2_PLACEMENT_3D('',#5213,#4255,#4256);
#3550=AXIS2_PLACEMENT_3D('',#5217,#4258,#4259);
#3551=AXIS2_PLACEMENT_3D('',#5219,#4260,#4261);
#3552=AXIS2_PLACEMENT_3D('',#5222,#4263,#4264);
#3553=AXIS2_PLACEMENT_3D('',#5223,#4265,#4266);
#3554=AXIS2_PLACEMENT_3D('',#5225,#4267,#4268);
#3555=AXIS2_PLACEMENT_3D('',#5227,#4270,#4271);
#3556=AXIS2_PLACEMENT_3D('',#5234,#4276,#4277);
#3557=AXIS2_PLACEMENT_3D('',#5236,#4279,#4280);
#3558=AXIS2_PLACEMENT_3D('',#5243,#4285,#4286);
#3559=AXIS2_PLACEMENT_3D('',#5244,#4287,#4288);
#3560=AXIS2_PLACEMENT_3D('',#5245,#4289,#4290);
#3561=AXIS2_PLACEMENT_3D('',#5246,#4291,#4292);
#3562=AXIS2_PLACEMENT_3D('',#5250,#4295,#4296);
#3563=AXIS2_PLACEMENT_3D('',#5254,#4299,#4300);
#3564=AXIS2_PLACEMENT_3D('',#5256,#4302,#4303);
#3565=AXIS2_PLACEMENT_3D('',#5257,#4304,#4305);
#3566=AXIS2_PLACEMENT_3D('',#5261,#4308,#4309);
#3567=AXIS2_PLACEMENT_3D('',#5265,#4312,#4313);
#3568=AXIS2_PLACEMENT_3D('',#5267,#4315,#4316);
#3569=AXIS2_PLACEMENT_3D('',#5268,#4317,#4318);
#3570=AXIS2_PLACEMENT_3D('',#5270,#4320,#4321);
#3571=AXIS2_PLACEMENT_3D('',#5272,#4323,#4324);
#3572=AXIS2_PLACEMENT_3D('',#5273,#4325,#4326);
#3573=AXIS2_PLACEMENT_3D('',#5275,#4328,#4329);
#3574=AXIS2_PLACEMENT_3D('',#5277,#4331,#4332);
#4139=DIRECTION('axis',(0.,0.,1.));
#4140=DIRECTION('refdir',(1.,0.,0.));
#4141=DIRECTION('center_axis',(-1.22464679914735E-16,0.,1.));
#4142=DIRECTION('ref_axis',(-1.,0.,-1.22464679914735E-16));
#4143=DIRECTION('',(-1.,1.32329071915687E-32,-2.28847549044393E-17));
#4144=DIRECTION('',(4.88654500275157E-16,1.,5.98429169650921E-32));
#4145=DIRECTION('center_axis',(1.22464679914735E-16,0.,-1.));
#4146=DIRECTION('ref_axis',(0.,-1.,0.));
#4147=DIRECTION('',(1.,-4.88654500275157E-16,1.22464679914735E-16));
#4148=DIRECTION('center_axis',(1.22464679914735E-16,0.,-1.));
#4149=DIRECTION('ref_axis',(0.,-1.,0.));
#4150=DIRECTION('',(4.88654500275157E-16,1.,5.9842916965092E-32));
#4151=DIRECTION('',(-1.,1.32329071915687E-32,-2.28847549044393E-17));
#4152=DIRECTION('',(5.78241158658936E-16,1.,7.08141184086923E-32));
#4153=DIRECTION('center_axis',(1.22464679914735E-16,0.,-1.));
#4154=DIRECTION('ref_axis',(0.,-1.,0.));
#4155=DIRECTION('',(1.,-5.78241158658936E-16,1.22464679914735E-16));
#4156=DIRECTION('center_axis',(1.22464679914735E-16,0.,-1.));
#4157=DIRECTION('ref_axis',(0.,-1.,0.));
#4158=DIRECTION('',(5.78241158658936E-16,1.,7.08141184086923E-32));
#4159=DIRECTION('center_axis',(-1.22464679914735E-16,0.,1.));
#4160=DIRECTION('ref_axis',(-1.,0.,-1.22464679914735E-16));
#4161=DIRECTION('',(5.78241158658936E-16,1.,7.08141184086923E-32));
#4162=DIRECTION('center_axis',(1.22464679914735E-16,0.,-1.));
#4163=DIRECTION('ref_axis',(0.,-1.,0.));
#4164=DIRECTION('',(1.,-5.78241158658936E-16,1.22464679914735E-16));
#4165=DIRECTION('center_axis',(1.22464679914735E-16,0.,-1.));
#4166=DIRECTION('ref_axis',(0.,-1.,0.));
#4167=DIRECTION('',(5.78241158658936E-16,1.,7.08141184086923E-32));
#4168=DIRECTION('',(-1.,1.32329071915687E-32,-2.28847549044393E-17));
#4169=DIRECTION('',(4.88654500275157E-16,1.,5.9842916965092E-32));
#4170=DIRECTION('center_axis',(1.22464679914735E-16,0.,-1.));
#4171=DIRECTION('ref_axis',(0.,-1.,0.));
#4172=DIRECTION('',(1.,0.,1.22464679914735E-16));
#4173=DIRECTION('center_axis',(1.22464679914735E-16,0.,-1.));
#4174=DIRECTION('ref_axis',(0.,-1.,0.));
#4175=DIRECTION('',(4.88654500275157E-16,1.,5.98429169650921E-32));
#4176=DIRECTION('',(-1.,1.32329071915687E-32,-2.28847549044393E-17));
#4177=DIRECTION('center_axis',(-5.78241158658936E-16,-1.,-7.08141184086922E-32));
#4178=DIRECTION('ref_axis',(1.,-5.78241158658936E-16,0.));
#4179=DIRECTION('',(-4.09476378780532E-47,-7.08141184086922E-32,1.));
#4180=DIRECTION('',(-1.,5.78241158658936E-16,4.09476378780532E-47));
#4181=DIRECTION('',(-1.22464679914735E-16,0.,1.));
#4182=DIRECTION('',(-1.22464679914735E-16,0.,1.));
#4183=DIRECTION('',(-1.,5.78241158658936E-16,-3.06161699786839E-16));
#4184=DIRECTION('',(-1.22464679914735E-16,0.,1.));
#4185=DIRECTION('',(-1.,5.78241158658936E-16,4.09476378780532E-47));
#4186=DIRECTION('center_axis',(-1.22464679914735E-16,0.,1.));
#4187=DIRECTION('ref_axis',(-1.,0.,-1.22464679914735E-16));
#4188=DIRECTION('center_axis',(3.06161699786839E-16,0.,-1.));
#4189=DIRECTION('ref_axis',(-1.,0.,-3.06161699786839E-16));
#4190=DIRECTION('',(-1.22464679914735E-16,0.,1.));
#4191=DIRECTION('center_axis',(0.,-7.08141184086922E-32,1.));
#4192=DIRECTION('ref_axis',(0.,-1.,-7.08141184086922E-32));
#4193=DIRECTION('center_axis',(-1.,5.78241158658936E-16,-1.22464679914735E-16));
#4194=DIRECTION('ref_axis',(-5.78241158658936E-16,-1.,-1.41228329145101E-48));
#4195=DIRECTION('',(5.78241158658936E-16,1.,1.77035296021731E-31));
#4196=DIRECTION('',(-1.22464679914735E-16,0.,1.));
#4197=DIRECTION('',(-5.78241158658936E-16,-1.,0.));
#4198=DIRECTION('',(1.22464679914735E-16,-7.08141184086923E-32,-1.));
#4199=DIRECTION('',(-5.78241158658936E-16,-1.,0.));
#4200=DIRECTION('',(-1.22464679914735E-16,0.,1.));
#4201=DIRECTION('',(-2.28847549044393E-17,-5.78241158658936E-16,1.));
#4202=DIRECTION('',(1.32329071915687E-32,-1.,-5.78241158658936E-16));
#4203=DIRECTION('',(-2.28847549044393E-17,-5.78241158658936E-16,1.));
#4204=DIRECTION('',(-1.22464679914735E-16,0.,1.));
#4205=DIRECTION('',(5.78241158658936E-16,1.,7.08141184086922E-32));
#4206=DIRECTION('',(1.22464679914735E-16,-1.09476442525376E-47,-1.));
#4207=DIRECTION('',(5.78241158658936E-16,1.,7.08141184086922E-32));
#4208=DIRECTION('center_axis',(-1.22464679914735E-16,0.,1.));
#4209=DIRECTION('ref_axis',(-1.,0.,-1.22464679914735E-16));
#4210=DIRECTION('',(-1.22464679914735E-16,0.,1.));
#4211=DIRECTION('center_axis',(0.,0.,-1.));
#4212=DIRECTION('ref_axis',(-1.,0.,0.));
#4213=DIRECTION('center_axis',(-1.,4.88654500275157E-16,-1.22464679914735E-16));
#4214=DIRECTION('ref_axis',(-4.88654500275157E-16,-1.,-3.23663765428249E-48));
#4215=DIRECTION('',(-1.22464679914735E-16,0.,1.));
#4216=DIRECTION('',(-2.28847549044393E-17,-5.78241158658936E-16,1.));
#4217=DIRECTION('',(1.32329071915687E-32,-1.,-5.78241158658936E-16));
#4218=DIRECTION('',(-2.28847549044393E-17,-5.78241158658936E-16,1.));
#4219=DIRECTION('',(-1.22464679914735E-16,0.,1.));
#4220=DIRECTION('',(4.88654500275157E-16,1.,1.4960729241273E-31));
#4221=DIRECTION('center_axis',(-1.22464679914735E-16,0.,1.));
#4222=DIRECTION('ref_axis',(-1.,0.,-1.22464679914735E-16));
#4223=DIRECTION('',(-1.22464679914735E-16,0.,1.));
#4224=DIRECTION('center_axis',(3.06161699786839E-16,0.,-1.));
#4225=DIRECTION('ref_axis',(-1.,0.,-3.06161699786839E-16));
#4226=DIRECTION('center_axis',(-4.88654500275157E-16,-1.,-5.9842916965092E-32));
#4227=DIRECTION('ref_axis',(1.,-4.88654500275157E-16,0.));
#4228=DIRECTION('',(-1.22464679914735E-16,0.,1.));
#4229=DIRECTION('',(1.,-4.88654500275157E-16,3.06161699786839E-16));
#4230=DIRECTION('center_axis',(-1.22464679914735E-16,0.,1.));
#4231=DIRECTION('ref_axis',(-1.,0.,-1.22464679914735E-16));
#4232=DIRECTION('',(-1.22464679914735E-16,0.,1.));
#4233=DIRECTION('center_axis',(3.06161699786839E-16,0.,-1.));
#4234=DIRECTION('ref_axis',(-1.,0.,-3.06161699786839E-16));
#4235=DIRECTION('center_axis',(1.,-4.88654500275157E-16,1.22464679914735E-16));
#4236=DIRECTION('ref_axis',(4.88654500275157E-16,1.,3.23663765428249E-48));
#4237=DIRECTION('',(-1.22464679914735E-16,0.,1.));
#4238=DIRECTION('',(-2.28847549044393E-17,-5.78241158658936E-16,1.));
#4239=DIRECTION('',(1.32329071915687E-32,-1.,-5.78241158658936E-16));
#4240=DIRECTION('',(-2.28847549044393E-17,-5.78241158658936E-16,1.));
#4241=DIRECTION('',(4.88654500275157E-16,1.,1.4960729241273E-31));
#4242=DIRECTION('center_axis',(-1.22464679914735E-16,0.,1.));
#4243=DIRECTION('ref_axis',(-1.,0.,-1.22464679914735E-16));
#4244=DIRECTION('',(-1.22464679914735E-16,0.,1.));
#4245=DIRECTION('center_axis',(3.06161699786839E-16,0.,-1.));
#4246=DIRECTION('ref_axis',(-1.,0.,-3.06161699786839E-16));
#4247=DIRECTION('center_axis',(0.,1.,0.));
#4248=DIRECTION('ref_axis',(0.,0.,-1.));
#4249=DIRECTION('',(-1.22464679914735E-16,0.,1.));
#4250=DIRECTION('',(1.,0.,3.06161699786839E-16));
#4251=DIRECTION('center_axis',(-1.22464679914735E-16,0.,1.));
#4252=DIRECTION('ref_axis',(-1.,0.,-1.22464679914735E-16));
#4253=DIRECTION('center_axis',(3.06161699786839E-16,0.,-1.));
#4254=DIRECTION('ref_axis',(-1.,0.,-3.06161699786839E-16));
#4255=DIRECTION('center_axis',(-3.06161699786839E-16,0.,1.));
#4256=DIRECTION('ref_axis',(1.,0.,3.06161699786839E-16));
#4257=DIRECTION('',(1.,-5.78241158658936E-16,3.06161699786839E-16));
#4258=DIRECTION('center_axis',(3.06161699786839E-16,0.,-1.));
#4259=DIRECTION('ref_axis',(-1.,0.,-3.06161699786839E-16));
#4260=DIRECTION('center_axis',(3.06161699786839E-16,0.,-1.));
#4261=DIRECTION('ref_axis',(-1.,0.,-3.06161699786839E-16));
#4262=DIRECTION('',(-5.78241158658936E-16,-1.,-1.77035296021731E-31));
#4263=DIRECTION('center_axis',(3.06161699786839E-16,0.,-1.));
#4264=DIRECTION('ref_axis',(-1.,0.,-3.06161699786839E-16));
#4265=DIRECTION('center_axis',(-1.22464679914735E-16,0.,1.));
#4266=DIRECTION('ref_axis',(-1.,0.,-1.22464679914735E-16));
#4267=DIRECTION('center_axis',(0.,0.,-1.));
#4268=DIRECTION('ref_axis',(-1.,0.,0.));
#4269=DIRECTION('',(-1.22464679914735E-16,0.,1.));
#4270=DIRECTION('center_axis',(5.78241158658936E-16,1.,7.08141184086922E-32));
#4271=DIRECTION('ref_axis',(-1.,5.78241158658936E-16,0.));
#4272=DIRECTION('',(-1.,5.78241158658936E-16,0.));
#4273=DIRECTION('',(-1.22464679914735E-16,0.,1.));
#4274=DIRECTION('',(-1.,5.78241158658936E-16,0.));
#4275=DIRECTION('',(0.,0.,1.));
#4276=DIRECTION('center_axis',(-1.22464679914735E-16,0.,1.));
#4277=DIRECTION('ref_axis',(-1.,0.,-1.22464679914735E-16));
#4278=DIRECTION('',(-1.22464679914735E-16,0.,1.));
#4279=DIRECTION('center_axis',(1.,-5.78241158658936E-16,1.22464679914735E-16));
#4280=DIRECTION('ref_axis',(5.78241158658936E-16,1.,1.41228329145101E-48));
#4281=DIRECTION('',(-1.22464679914735E-16,0.,1.));
#4282=DIRECTION('',(-2.28847549044393E-17,-5.78241158658936E-16,1.));
#4283=DIRECTION('',(1.32329071915687E-32,-1.,-5.78241158658936E-16));
#4284=DIRECTION('',(-2.28847549044393E-17,-5.78241158658936E-16,1.));
#4285=DIRECTION('center_axis',(-1.22464679914735E-16,0.,1.));
#4286=DIRECTION('ref_axis',(-1.,0.,-1.22464679914735E-16));
#4287=DIRECTION('center_axis',(-1.22464679914735E-16,0.,1.));
#4288=DIRECTION('ref_axis',(-1.,0.,-1.22464679914735E-16));
#4289=DIRECTION('center_axis',(0.,-7.08141184086922E-32,1.));
#4290=DIRECTION('ref_axis',(0.,-1.,-7.08141184086922E-32));
#4291=DIRECTION('center_axis',(0.,0.,1.));
#4292=DIRECTION('ref_axis',(-1.,0.,0.));
#4293=DIRECTION('',(5.78241158658936E-16,1.,0.));
#4294=DIRECTION('',(-1.,5.78241158658936E-16,0.));
#4295=DIRECTION('center_axis',(1.,-5.78241158658936E-16,0.));
#4296=DIRECTION('ref_axis',(5.78241158658936E-16,1.,0.));
#4297=DIRECTION('',(5.78241158658936E-16,1.,0.));
#4298=DIRECTION('',(0.,0.,1.));
#4299=DIRECTION('center_axis',(0.,0.,1.));
#4300=DIRECTION('ref_axis',(-1.,0.,0.));
#4301=DIRECTION('',(-1.,5.78241158658936E-16,0.));
#4302=DIRECTION('center_axis',(-5.78241158658936E-16,-1.,0.));
#4303=DIRECTION('ref_axis',(1.,-5.78241158658936E-16,0.));
#4304=DIRECTION('center_axis',(0.,7.08141184086922E-32,-1.));
#4305=DIRECTION('ref_axis',(0.,-1.,-7.08141184086922E-32));
#4306=DIRECTION('',(-1.,5.78241158658936E-16,4.09476378780532E-47));
#4307=DIRECTION('',(-5.78241158658936E-16,-1.,-7.08141184086922E-32));
#4308=DIRECTION('center_axis',(-1.,5.78241158658936E-16,0.));
#4309=DIRECTION('ref_axis',(-5.78241158658936E-16,-1.,0.));
#4310=DIRECTION('',(-4.09476378780532E-47,-7.08141184086922E-32,1.));
#4311=DIRECTION('',(-5.78241158658936E-16,-1.,-7.08141184086922E-32));
#4312=DIRECTION('center_axis',(0.,7.08141184086922E-32,-1.));
#4313=DIRECTION('ref_axis',(0.,-1.,-7.08141184086922E-32));
#4314=DIRECTION('',(-1.,5.78241158658936E-16,4.09476378780532E-47));
#4315=DIRECTION('center_axis',(-5.78241158658936E-16,-1.,-7.08141184086922E-32));
#4316=DIRECTION('ref_axis',(1.,-5.78241158658936E-16,-4.09476378780532E-47));
#4317=DIRECTION('center_axis',(1.78184314006146E-48,-1.,-5.78241158658936E-16));
#4318=DIRECTION('ref_axis',(-6.41902719210046E-80,-5.78241158658936E-16,
1.));
#4319=DIRECTION('',(-1.,1.32329071915687E-32,-2.28847549044393E-17));
#4320=DIRECTION('center_axis',(1.78184314006146E-48,-1.,-5.78241158658936E-16));
#4321=DIRECTION('ref_axis',(-6.41902719210046E-80,-5.78241158658936E-16,
1.));
#4322=DIRECTION('',(-1.,1.32329071915687E-32,-2.28847549044393E-17));
#4323=DIRECTION('center_axis',(-2.28847549044393E-17,-5.78241158658936E-16,
1.));
#4324=DIRECTION('ref_axis',(1.,-1.32329071915687E-32,2.28847549044393E-17));
#4325=DIRECTION('center_axis',(1.78184314006146E-48,-1.,-5.78241158658936E-16));
#4326=DIRECTION('ref_axis',(-6.41902719210046E-80,-5.78241158658936E-16,
1.));
#4327=DIRECTION('',(-1.,1.32329071915687E-32,-2.28847549044393E-17));
#4328=DIRECTION('center_axis',(1.78184314006146E-48,-1.,-5.78241158658936E-16));
#4329=DIRECTION('ref_axis',(-6.41902719210046E-80,-5.78241158658936E-16,
1.));
#4330=DIRECTION('',(-1.,1.32329071915687E-32,-2.28847549044393E-17));
#4331=DIRECTION('center_axis',(-2.28847549044393E-17,-5.78241158658936E-16,
1.));
#4332=DIRECTION('ref_axis',(1.,-1.32329071915687E-32,2.28847549044393E-17));
#5072=CARTESIAN_POINT('',(0.,0.,0.));
#5073=CARTESIAN_POINT('Origin',(-360.,850.,-2152.));
#5074=CARTESIAN_POINT('',(-340.,855.,-2152.));
#5075=CARTESIAN_POINT('',(-344.,855.,-2152.));
#5076=CARTESIAN_POINT('',(-342.,855.,-2152.));
#5077=CARTESIAN_POINT('',(-344.,864.2,-2152.));
#5078=CARTESIAN_POINT('',(-344.,850.,-2152.));
#5079=CARTESIAN_POINT('',(-345.8,866.,-2152.));
#5080=CARTESIAN_POINT('Origin',(-345.8,864.2,-2152.));
#5081=CARTESIAN_POINT('',(-374.2,866.,-2152.));
#5082=CARTESIAN_POINT('',(-360.,866.,-2152.));
#5083=CARTESIAN_POINT('',(-376.,864.2,-2152.));
#5084=CARTESIAN_POINT('Origin',(-374.2,864.2,-2152.));
#5085=CARTESIAN_POINT('',(-376.,855.,-2152.));
#5086=CARTESIAN_POINT('',(-376.,850.,-2152.));
#5087=CARTESIAN_POINT('',(-380.,855.,-2152.));
#5088=CARTESIAN_POINT('',(-378.,855.,-2152.));
#5089=CARTESIAN_POINT('',(-380.,868.,-2152.));
#5090=CARTESIAN_POINT('',(-380.,850.,-2152.));
#5091=CARTESIAN_POINT('',(-378.,870.,-2152.));
#5092=CARTESIAN_POINT('Origin',(-378.,868.,-2152.));
#5093=CARTESIAN_POINT('',(-342.,870.,-2152.));
#5094=CARTESIAN_POINT('',(-360.,870.,-2152.));
#5095=CARTESIAN_POINT('',(-340.,868.,-2152.));
#5096=CARTESIAN_POINT('Origin',(-342.,868.,-2152.));
#5097=CARTESIAN_POINT('',(-340.,850.,-2152.));
#5098=CARTESIAN_POINT('Origin',(-360.,850.,-2152.));
#5099=CARTESIAN_POINT('',(-340.,845.,-2152.));
#5100=CARTESIAN_POINT('',(-340.,832.,-2152.));
#5101=CARTESIAN_POINT('',(-340.,850.,-2152.));
#5102=CARTESIAN_POINT('',(-342.,830.,-2152.));
#5103=CARTESIAN_POINT('Origin',(-342.,832.,-2152.));
#5104=CARTESIAN_POINT('',(-378.,830.,-2152.));
#5105=CARTESIAN_POINT('',(-360.,830.,-2152.));
#5106=CARTESIAN_POINT('',(-380.,832.,-2152.));
#5107=CARTESIAN_POINT('Origin',(-378.,832.,-2152.));
#5108=CARTESIAN_POINT('',(-380.,845.,-2152.));
#5109=CARTESIAN_POINT('',(-380.,850.,-2152.));
#5110=CARTESIAN_POINT('',(-376.,845.,-2152.));
#5111=CARTESIAN_POINT('',(-378.,845.,-2152.));
#5112=CARTESIAN_POINT('',(-376.,835.8,-2152.));
#5113=CARTESIAN_POINT('',(-376.,850.,-2152.));
#5114=CARTESIAN_POINT('',(-374.2,834.,-2152.));
#5115=CARTESIAN_POINT('Origin',(-374.2,835.8,-2152.));
#5116=CARTESIAN_POINT('',(-345.8,834.,-2152.));
#5117=CARTESIAN_POINT('',(-360.,834.,-2152.));
#5118=CARTESIAN_POINT('',(-344.,835.8,-2152.));
#5119=CARTESIAN_POINT('Origin',(-345.8,835.8,-2152.));
#5120=CARTESIAN_POINT('',(-344.,845.,-2152.));
#5121=CARTESIAN_POINT('',(-344.,850.,-2152.));
#5122=CARTESIAN_POINT('',(-342.,845.,-2152.));
#5123=CARTESIAN_POINT('Origin',(-360.,830.,-2152.));
#5124=CARTESIAN_POINT('',(-375.,830.,-1958.));
#5125=CARTESIAN_POINT('',(-375.,830.,-1946.));
#5126=CARTESIAN_POINT('',(-375.,830.,-1952.));
#5127=CARTESIAN_POINT('',(-378.,830.,-1958.));
#5128=CARTESIAN_POINT('',(-378.,830.,-1958.));
#5129=CARTESIAN_POINT('',(-378.,830.,-2152.));
#5130=CARTESIAN_POINT('',(-342.,830.,-172.));
#5131=CARTESIAN_POINT('',(-342.,830.,-2152.));
#5132=CARTESIAN_POINT('',(-378.,830.,-172.));
#5133=CARTESIAN_POINT('',(-360.,830.,-172.));
#5134=CARTESIAN_POINT('',(-378.,830.,-1946.));
#5135=CARTESIAN_POINT('',(-378.,830.,-2152.));
#5136=CARTESIAN_POINT('',(-378.,830.,-1946.));
#5137=CARTESIAN_POINT('Origin',(-378.,832.,-2152.));
#5138=CARTESIAN_POINT('',(-380.,832.,-172.));
#5139=CARTESIAN_POINT('Origin',(-378.,832.,-172.));
#5140=CARTESIAN_POINT('',(-380.,832.,-1946.));
#5141=CARTESIAN_POINT('',(-380.,832.,-2152.));
#5142=CARTESIAN_POINT('Origin',(-378.,832.,-1946.));
#5143=CARTESIAN_POINT('Origin',(-380.,850.,-2152.));
#5144=CARTESIAN_POINT('',(-380.,868.,-172.));
#5145=CARTESIAN_POINT('',(-380.,850.,-172.));
#5146=CARTESIAN_POINT('',(-380.,868.,-1946.));
#5147=CARTESIAN_POINT('',(-380.,868.,-2152.));
#5148=CARTESIAN_POINT('',(-380.,867.,-1946.));
#5149=CARTESIAN_POINT('',(-380.,850.,-1946.));
#5150=CARTESIAN_POINT('',(-380.,867.,-1958.));
#5151=CARTESIAN_POINT('',(-380.,867.,-2152.));
#5152=CARTESIAN_POINT('',(-380.,868.,-1958.));
#5153=CARTESIAN_POINT('',(-380.,850.,-1958.));
#5154=CARTESIAN_POINT('',(-380.,868.,-2152.));
#5155=CARTESIAN_POINT('',(-380.,855.,-2155.));
#5156=CARTESIAN_POINT('',(-380.,855.,-2155.));
#5157=CARTESIAN_POINT('',(-380.,845.,-2155.));
#5158=CARTESIAN_POINT('',(-380.,850.,-2155.));
#5159=CARTESIAN_POINT('',(-380.,845.,-2155.));
#5160=CARTESIAN_POINT('',(-380.,832.,-1958.));
#5161=CARTESIAN_POINT('',(-380.,832.,-2152.));
#5162=CARTESIAN_POINT('',(-380.,834.,-1958.));
#5163=CARTESIAN_POINT('',(-380.,850.,-1958.));
#5164=CARTESIAN_POINT('',(-380.,834.,-1946.));
#5165=CARTESIAN_POINT('',(-380.,834.,-2152.));
#5166=CARTESIAN_POINT('',(-380.,850.,-1946.));
#5167=CARTESIAN_POINT('Origin',(-378.,868.,-2152.));
#5168=CARTESIAN_POINT('',(-378.,870.,-1958.));
#5169=CARTESIAN_POINT('',(-378.,870.,-2152.));
#5170=CARTESIAN_POINT('Origin',(-378.,868.,-1958.));
#5171=CARTESIAN_POINT('Origin',(-344.,850.,-2152.));
#5172=CARTESIAN_POINT('',(-344.,864.2,-172.));
#5173=CARTESIAN_POINT('',(-344.,864.2,-2152.));
#5174=CARTESIAN_POINT('',(-344.,855.,-2155.));
#5175=CARTESIAN_POINT('',(-344.,855.,-2155.));
#5176=CARTESIAN_POINT('',(-344.,845.,-2155.));
#5177=CARTESIAN_POINT('',(-344.,850.,-2155.));
#5178=CARTESIAN_POINT('',(-344.,845.,-2155.));
#5179=CARTESIAN_POINT('',(-344.,835.8,-172.));
#5180=CARTESIAN_POINT('',(-344.,835.8,-2152.));
#5181=CARTESIAN_POINT('',(-344.,850.,-172.));
#5182=CARTESIAN_POINT('Origin',(-345.8,864.2,-2152.));
#5183=CARTESIAN_POINT('',(-345.8,866.,-172.));
#5184=CARTESIAN_POINT('',(-345.8,866.,-2152.));
#5185=CARTESIAN_POINT('Origin',(-345.8,864.2,-172.));
#5186=CARTESIAN_POINT('Origin',(-360.,866.,-2152.));
#5187=CARTESIAN_POINT('',(-374.2,866.,-172.));
#5188=CARTESIAN_POINT('',(-374.2,866.,-2152.));
#5189=CARTESIAN_POINT('',(-360.,866.,-172.));
#5190=CARTESIAN_POINT('Origin',(-374.2,864.2,-2152.));
#5191=CARTESIAN_POINT('',(-376.,864.2,-172.));
#5192=CARTESIAN_POINT('',(-376.,864.2,-2152.));
#5193=CARTESIAN_POINT('Origin',(-374.2,864.2,-172.));
#5194=CARTESIAN_POINT('Origin',(-376.,850.,-2152.));
#5195=CARTESIAN_POINT('',(-376.,835.8,-172.));
#5196=CARTESIAN_POINT('',(-376.,835.8,-2152.));
#5197=CARTESIAN_POINT('',(-376.,845.,-2155.));
#5198=CARTESIAN_POINT('',(-376.,845.,-2155.));
#5199=CARTESIAN_POINT('',(-376.,855.,-2155.));
#5200=CARTESIAN_POINT('',(-376.,850.,-2155.));
#5201=CARTESIAN_POINT('',(-376.,855.,-2155.));
#5202=CARTESIAN_POINT('',(-376.,850.,-172.));
#5203=CARTESIAN_POINT('Origin',(-374.2,835.8,-2152.));
#5204=CARTESIAN_POINT('',(-374.2,834.,-172.));
#5205=CARTESIAN_POINT('',(-374.2,834.,-2152.));
#5206=CARTESIAN_POINT('Origin',(-374.2,835.8,-172.));
#5207=CARTESIAN_POINT('Origin',(-360.,834.,-2152.));
#5208=CARTESIAN_POINT('',(-345.8,834.,-172.));
#5209=CARTESIAN_POINT('',(-345.8,834.,-2152.));
#5210=CARTESIAN_POINT('',(-360.,834.,-172.));
#5211=CARTESIAN_POINT('Origin',(-345.8,835.8,-2152.));
#5212=CARTESIAN_POINT('Origin',(-345.8,835.8,-172.));
#5213=CARTESIAN_POINT('Origin',(-360.,850.,-172.));
#5214=CARTESIAN_POINT('',(-378.,870.,-172.));
#5215=CARTESIAN_POINT('',(-342.,870.,-172.));
#5216=CARTESIAN_POINT('',(-360.,870.,-172.));
#5217=CARTESIAN_POINT('Origin',(-378.,868.,-172.));
#5218=CARTESIAN_POINT('',(-340.,832.,-172.));
#5219=CARTESIAN_POINT('Origin',(-342.,832.,-172.));
#5220=CARTESIAN_POINT('',(-340.,868.,-172.));
#5221=CARTESIAN_POINT('',(-340.,850.,-172.));
#5222=CARTESIAN_POINT('Origin',(-342.,868.,-172.));
#5223=CARTESIAN_POINT('Origin',(-378.,868.,-2152.));
#5224=CARTESIAN_POINT('',(-378.,870.,-1946.));
#5225=CARTESIAN_POINT('Origin',(-378.,868.,-1946.));
#5226=CARTESIAN_POINT('',(-378.,870.,-2152.));
#5227=CARTESIAN_POINT('Origin',(-360.,870.,-2152.));
#5228=CARTESIAN_POINT('',(-375.,870.,-1946.));
#5229=CARTESIAN_POINT('',(-378.,870.,-1946.));
#5230=CARTESIAN_POINT('',(-342.,870.,-2152.));
#5231=CARTESIAN_POINT('',(-375.,870.,-1958.));
#5232=CARTESIAN_POINT('',(-378.,870.,-1958.));
#5233=CARTESIAN_POINT('',(-375.,870.,-1952.));
#5234=CARTESIAN_POINT('Origin',(-342.,868.,-2152.));
#5235=CARTESIAN_POINT('',(-340.,868.,-2152.));
#5236=CARTESIAN_POINT('Origin',(-340.,850.,-2152.));
#5237=CARTESIAN_POINT('',(-340.,832.,-2152.));
#5238=CARTESIAN_POINT('',(-340.,845.,-2155.));
#5239=CARTESIAN_POINT('',(-340.,845.,-2155.));
#5240=CARTESIAN_POINT('',(-340.,855.,-2155.));
#5241=CARTESIAN_POINT('',(-340.,850.,-2155.));
#5242=CARTESIAN_POINT('',(-340.,855.,-2155.));
#5243=CARTESIAN_POINT('Origin',(-342.,832.,-2152.));
#5244=CARTESIAN_POINT('Origin',(-378.,832.,-2152.));
#5245=CARTESIAN_POINT('Origin',(-378.,832.,-1958.));
#5246=CARTESIAN_POINT('Origin',(-378.,867.,-1946.));
#5247=CARTESIAN_POINT('',(-375.,867.,-1946.));
#5248=CARTESIAN_POINT('',(-375.,867.,-1946.));
#5249=CARTESIAN_POINT('',(-378.,867.,-1946.));
#5250=CARTESIAN_POINT('Origin',(-375.,867.,-1952.));
#5251=CARTESIAN_POINT('',(-375.,867.,-1958.));
#5252=CARTESIAN_POINT('',(-375.,867.,-1958.));
#5253=CARTESIAN_POINT('',(-375.,867.,-1952.));
#5254=CARTESIAN_POINT('Origin',(-378.,867.,-1958.));
#5255=CARTESIAN_POINT('',(-378.,867.,-1958.));
#5256=CARTESIAN_POINT('Origin',(-382.450381904372,867.,-1952.));
#5257=CARTESIAN_POINT('Origin',(-378.,834.,-1946.));
#5258=CARTESIAN_POINT('',(-375.,834.,-1946.));
#5259=CARTESIAN_POINT('',(-378.,834.,-1946.));
#5260=CARTESIAN_POINT('',(-375.,834.,-1946.));
#5261=CARTESIAN_POINT('Origin',(-375.,834.,-1952.));
#5262=CARTESIAN_POINT('',(-375.,834.,-1958.));
#5263=CARTESIAN_POINT('',(-375.,834.,-1952.));
#5264=CARTESIAN_POINT('',(-375.,834.,-1958.));
#5265=CARTESIAN_POINT('Origin',(-378.,834.,-1958.));
#5266=CARTESIAN_POINT('',(-378.,834.,-1958.));
#5267=CARTESIAN_POINT('Origin',(-382.450381904372,834.,-1952.));
#5268=CARTESIAN_POINT('Origin',(-378.,855.,-2155.));
#5269=CARTESIAN_POINT('',(-378.,855.,-2155.));
#5270=CARTESIAN_POINT('Origin',(-378.,845.,-2155.));
#5271=CARTESIAN_POINT('',(-378.,845.,-2155.));
#5272=CARTESIAN_POINT('Origin',(-360.,850.,-2155.));
#5273=CARTESIAN_POINT('Origin',(-342.,855.,-2155.));
#5274=CARTESIAN_POINT('',(-342.,855.,-2155.));
#5275=CARTESIAN_POINT('Origin',(-342.,845.,-2155.));
#5276=CARTESIAN_POINT('',(-342.,845.,-2155.));
#5277=CARTESIAN_POINT('Origin',(-360.,850.,-2155.));
#5493=UNCERTAINTY_MEASURE_WITH_UNIT(LENGTH_MEASURE(0.01),#5506,
'DISTANCE_ACCURACY_VALUE',
'Maximum model space distance between geometric entities at asserted c
onnectivities');
#5496=UNCERTAINTY_MEASURE_WITH_UNIT(LENGTH_MEASURE(0.01),#5506,
'DISTANCE_ACCURACY_VALUE',
'Maximum model space distance between geometric entities at asserted c
onnectivities');
#5502=(
GEOMETRIC_REPRESENTATION_CONTEXT(3)
GLOBAL_UNCERTAINTY_ASSIGNED_CONTEXT((#5493))
GLOBAL_UNIT_ASSIGNED_CONTEXT((#5506,#5508,#5509))
REPRESENTATION_CONTEXT('','3D')
);
#5505=(
GEOMETRIC_REPRESENTATION_CONTEXT(3)
GLOBAL_UNCERTAINTY_ASSIGNED_CONTEXT((#5496))
GLOBAL_UNIT_ASSIGNED_CONTEXT((#5506,#5508,#5509))
REPRESENTATION_CONTEXT('','3D')
);
#5506=(
LENGTH_UNIT()
NAMED_UNIT(*)
SI_UNIT(.MILLI.,.METRE.)
);
#5508=(
NAMED_UNIT(*)
PLANE_ANGLE_UNIT()
SI_UNIT($,.RADIAN.)
);
#5509=(
NAMED_UNIT(*)
SI_UNIT($,.STERADIAN.)
SOLID_ANGLE_UNIT()
);
#5515=SHAPE_DEFINITION_REPRESENTATION(#5523,#5541);
#5523=PRODUCT_DEFINITION_SHAPE('',$,#5550);
#5541=SHAPE_REPRESENTATION('',(#3519),#5502);
#5544=PRODUCT_DEFINITION_CONTEXT('part definition',#5570,'design');
#5550=PRODUCT_DEFINITION('Mast-third-vert-Mirrored',
'Mast-third-vert-Mirrored',#5558,#5544);
#5558=PRODUCT_DEFINITION_FORMATION('',$,#5577);
#5570=APPLICATION_CONTEXT(
'Core Data for Automotive Mechanical Design Process');
#5571=PRODUCT_CONTEXT('part definition',#5570,'mechanical');
#5577=PRODUCT('Mast-third-vert-Mirrored','Mast-third-vert-Mirrored',
'40x40x3mm-4pcs-mast-third-vert-Mirrored',(#5571));
#5585=PRESENTATION_STYLE_ASSIGNMENT((#5593));
#5593=SURFACE_STYLE_USAGE(.BOTH.,#5601);
#5601=SURFACE_SIDE_STYLE('',(#5609));
#5609=SURFACE_STYLE_FILL_AREA(#5617);
#5617=FILL_AREA_STYLE('Opaque(248,135,1)',(#5625));
#5625=FILL_AREA_STYLE_COLOUR('Opaque(248,135,1)',#5633);
#5633=COLOUR_RGB('Opaque(248,135,1)', 0.72549020, 0.75294118, 0.79215686);
ENDSEC;
END-ISO-10303-21;
